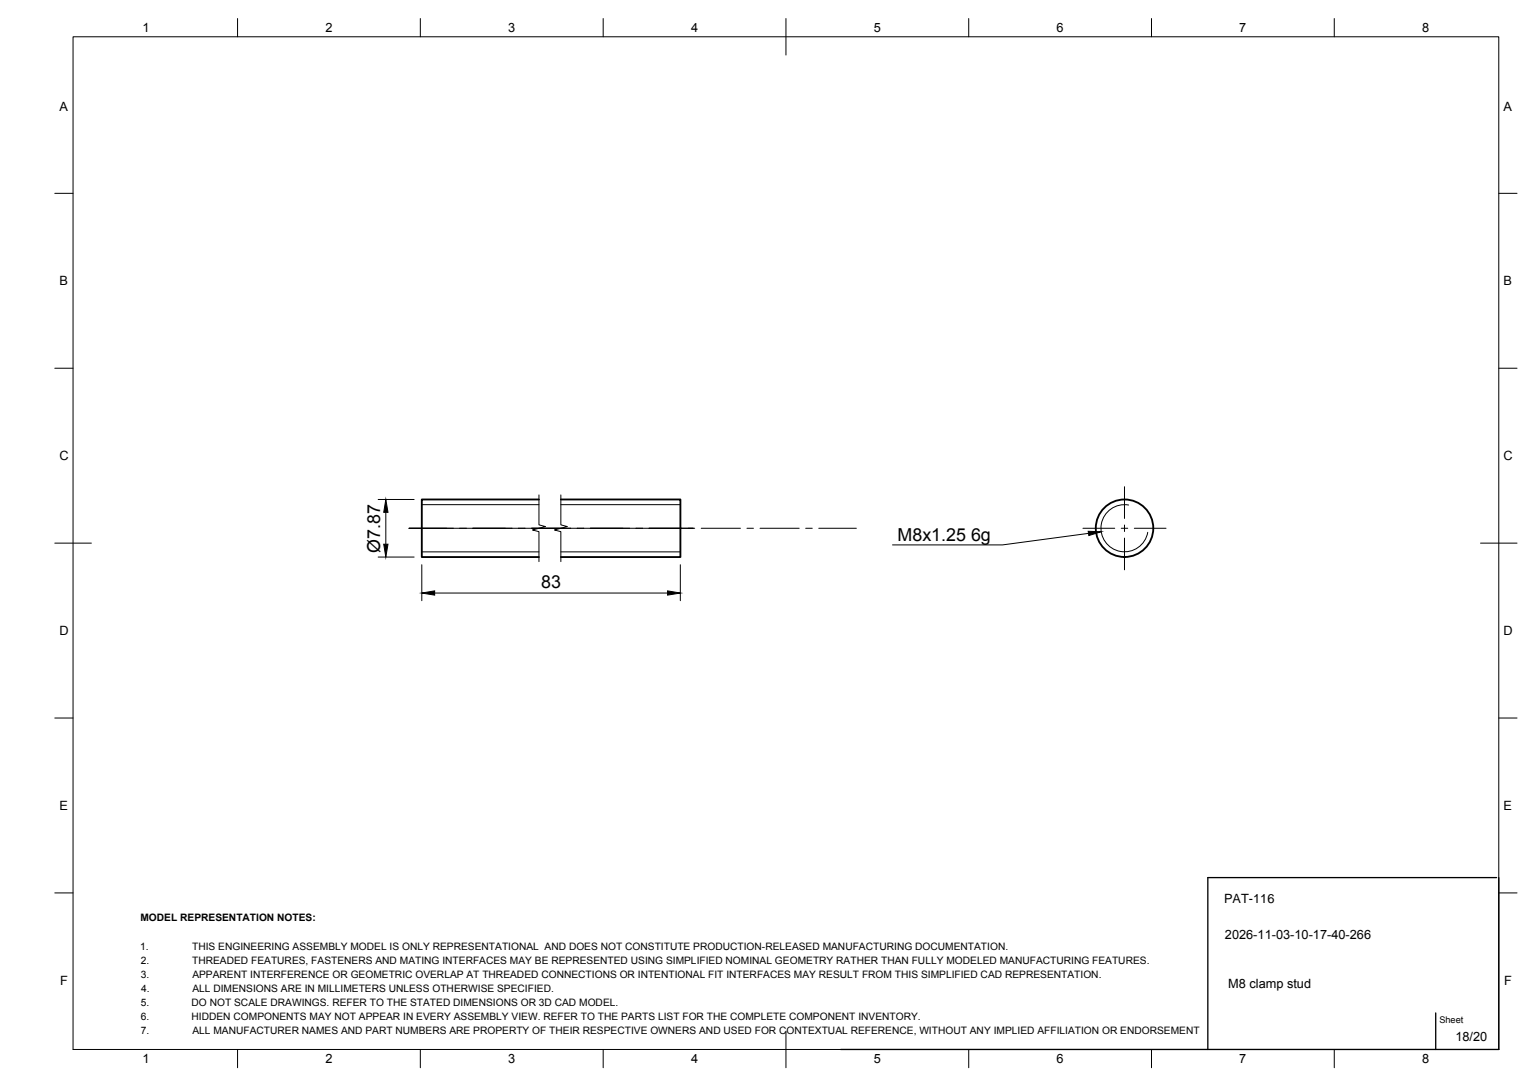
ISO-10303-21;
HEADER;
/* Generated by software containing ST-Developer
 * from STEP Tools, Inc. (www.steptools.com) 
 */

FILE_DESCRIPTION(
/* description */ ('V-block with clamp strap'),
/* implementation_level */ '2;1');

FILE_NAME(
/* name */ 'M8 clamp stud.step',
/* time_stamp */ '2026-10-27T10:50:53-07:00',
/* author */ (''),
/* organization */ (''),
/* preprocessor_version */ 'ST-DEVELOPER v20.2',
/* originating_system */ 'Autodesk Translation Framework v15.17.0.0',
/* authorisation */ '');

FILE_SCHEMA (('AUTOMOTIVE_DESIGN { 1 0 10303 214 3 1 1 }'));
ENDSEC;

DATA;
#10=MECHANICAL_DESIGN_GEOMETRIC_PRESENTATION_REPRESENTATION('',(#281),#7344);
#239=SHAPE_REPRESENTATION_RELATIONSHIP('SRR','None',#7458,#260);
#260=ADVANCED_BREP_SHAPE_REPRESENTATION('',(#300),#7337);
#281=STYLED_ITEM('',(#7638),#300);
#300=MANIFOLD_SOLID_BREP('Body1',#4165);
#484=CIRCLE('',#4759,0.3933);
#485=CIRCLE('',#4760,0.3933);
#554=CYLINDRICAL_SURFACE('',#4758,0.3933);
#762=FACE_OUTER_BOUND('',#1068,.T.);
#763=FACE_OUTER_BOUND('',#1069,.T.);
#764=FACE_OUTER_BOUND('',#1070,.T.);
#1068=EDGE_LOOP('',(#3600,#3601,#3602,#3603));
#1069=EDGE_LOOP('',(#3604));
#1070=EDGE_LOOP('',(#3605));
#1441=LINE('',#7094,#1806);
#1806=VECTOR('',#5883,0.4);
#2129=VERTEX_POINT('',#7091);
#2130=VERTEX_POINT('',#7093);
#2626=EDGE_CURVE('',#2129,#2129,#484,.F.);
#2627=EDGE_CURVE('',#2129,#2130,#1441,.T.);
#2628=EDGE_CURVE('',#2130,#2130,#485,.F.);
#3600=ORIENTED_EDGE('',*,*,#2626,.F.);
#3601=ORIENTED_EDGE('',*,*,#2627,.T.);
#3602=ORIENTED_EDGE('',*,*,#2628,.T.);
#3603=ORIENTED_EDGE('',*,*,#2627,.F.);
#3604=ORIENTED_EDGE('',*,*,#2626,.T.);
#3605=ORIENTED_EDGE('',*,*,#2628,.F.);
#3881=PLANE('',#4761);
#3882=PLANE('',#4762);
#4108=ADVANCED_FACE('',(#762),#554,.T.);
#4109=ADVANCED_FACE('',(#763),#3881,.T.);
#4110=ADVANCED_FACE('',(#764),#3882,.F.);
#4165=CLOSED_SHELL('',(#4108,#4109,#4110));
#4757=AXIS2_PLACEMENT_3D('',#7089,#5877,#5878);
#4758=AXIS2_PLACEMENT_3D('',#7090,#5879,#5880);
#4759=AXIS2_PLACEMENT_3D('',#7092,#5881,#5882);
#4760=AXIS2_PLACEMENT_3D('',#7095,#5884,#5885);
#4761=AXIS2_PLACEMENT_3D('',#7096,#5886,#5887);
#4762=AXIS2_PLACEMENT_3D('',#7097,#5888,#5889);
#5877=DIRECTION('axis',(0.,0.,1.));
#5878=DIRECTION('refdir',(1.,0.,0.));
#5879=DIRECTION('center_axis',(0.,0.,1.));
#5880=DIRECTION('ref_axis',(1.,0.,0.));
#5881=DIRECTION('center_axis',(0.,0.,-1.));
#5882=DIRECTION('ref_axis',(1.,0.,0.));
#5883=DIRECTION('',(0.,0.,-1.));
#5884=DIRECTION('center_axis',(0.,0.,-1.));
#5885=DIRECTION('ref_axis',(1.,0.,0.));
#5886=DIRECTION('center_axis',(0.,0.,1.));
#5887=DIRECTION('ref_axis',(1.,0.,0.));
#5888=DIRECTION('center_axis',(0.,0.,1.));
#5889=DIRECTION('ref_axis',(1.,0.,0.));
#7089=CARTESIAN_POINT('',(0.,0.,0.));
#7090=CARTESIAN_POINT('Origin',(10.,-4.,0.));
#7091=CARTESIAN_POINT('',(9.6067,-4.,8.3));
#7092=CARTESIAN_POINT('Origin',(10.,-4.,8.3));
#7093=CARTESIAN_POINT('',(9.6067,-4.,0.));
#7094=CARTESIAN_POINT('',(9.6067,-4.,0.));
#7095=CARTESIAN_POINT('Origin',(10.,-4.,0.));
#7096=CARTESIAN_POINT('Origin',(10.,-4.,8.3));
#7097=CARTESIAN_POINT('Origin',(10.,-4.,0.));
#7311=UNCERTAINTY_MEASURE_WITH_UNIT(LENGTH_MEASURE(0.001),#7345,
'DISTANCE_ACCURACY_VALUE',
'Maximum model space distance between geometric entities at asserted c
onnectivities');
#7318=UNCERTAINTY_MEASURE_WITH_UNIT(LENGTH_MEASURE(0.001),#7345,
'DISTANCE_ACCURACY_VALUE',
'Maximum model space distance between geometric entities at asserted c
onnectivities');
#7337=(
GEOMETRIC_REPRESENTATION_CONTEXT(3)
GLOBAL_UNCERTAINTY_ASSIGNED_CONTEXT((#7311))
GLOBAL_UNIT_ASSIGNED_CONTEXT((#7345,#7347,#7348))
REPRESENTATION_CONTEXT('','3D')
);
#7344=(
GEOMETRIC_REPRESENTATION_CONTEXT(3)
GLOBAL_UNCERTAINTY_ASSIGNED_CONTEXT((#7318))
GLOBAL_UNIT_ASSIGNED_CONTEXT((#7345,#7347,#7348))
REPRESENTATION_CONTEXT('','3D')
);
#7345=(
LENGTH_UNIT()
NAMED_UNIT(*)
SI_UNIT(.CENTI.,.METRE.)
);
#7347=(
NAMED_UNIT(*)
PLANE_ANGLE_UNIT()
SI_UNIT($,.RADIAN.)
);
#7348=(
NAMED_UNIT(*)
SI_UNIT($,.STERADIAN.)
SOLID_ANGLE_UNIT()
);
#7367=SHAPE_DEFINITION_REPRESENTATION(#7415,#7458);
#7415=PRODUCT_DEFINITION_SHAPE('',$,#7484);
#7458=SHAPE_REPRESENTATION('',(#4757),#7337);
#7465=PRODUCT_DEFINITION_CONTEXT('part definition',#7542,'design');
#7484=PRODUCT_DEFINITION('M8 clamp stud','M8 clamp stud',#7509,#7465);
#7509=PRODUCT_DEFINITION_FORMATION('',$,#7562);
#7542=APPLICATION_CONTEXT(
'Core Data for Automotive Mechanical Design Process');
#7543=PRODUCT_CONTEXT('part definition',#7542,'mechanical');
#7562=PRODUCT('M8 clamp stud','M8 clamp stud','M8 clamp stud',(#7543));
#7632=COLOUR_RGB('Black',0.12,0.14,0.17);
#7633=FILL_AREA_STYLE_COLOUR('',#7632);
#7634=FILL_AREA_STYLE('',(#7633));
#7635=SURFACE_STYLE_FILL_AREA(#7634);
#7636=SURFACE_SIDE_STYLE('',(#7635));
#7637=SURFACE_STYLE_USAGE(.BOTH.,#7636);
#7638=PRESENTATION_STYLE_ASSIGNMENT((#7637));
ENDSEC;
END-ISO-10303-21;
